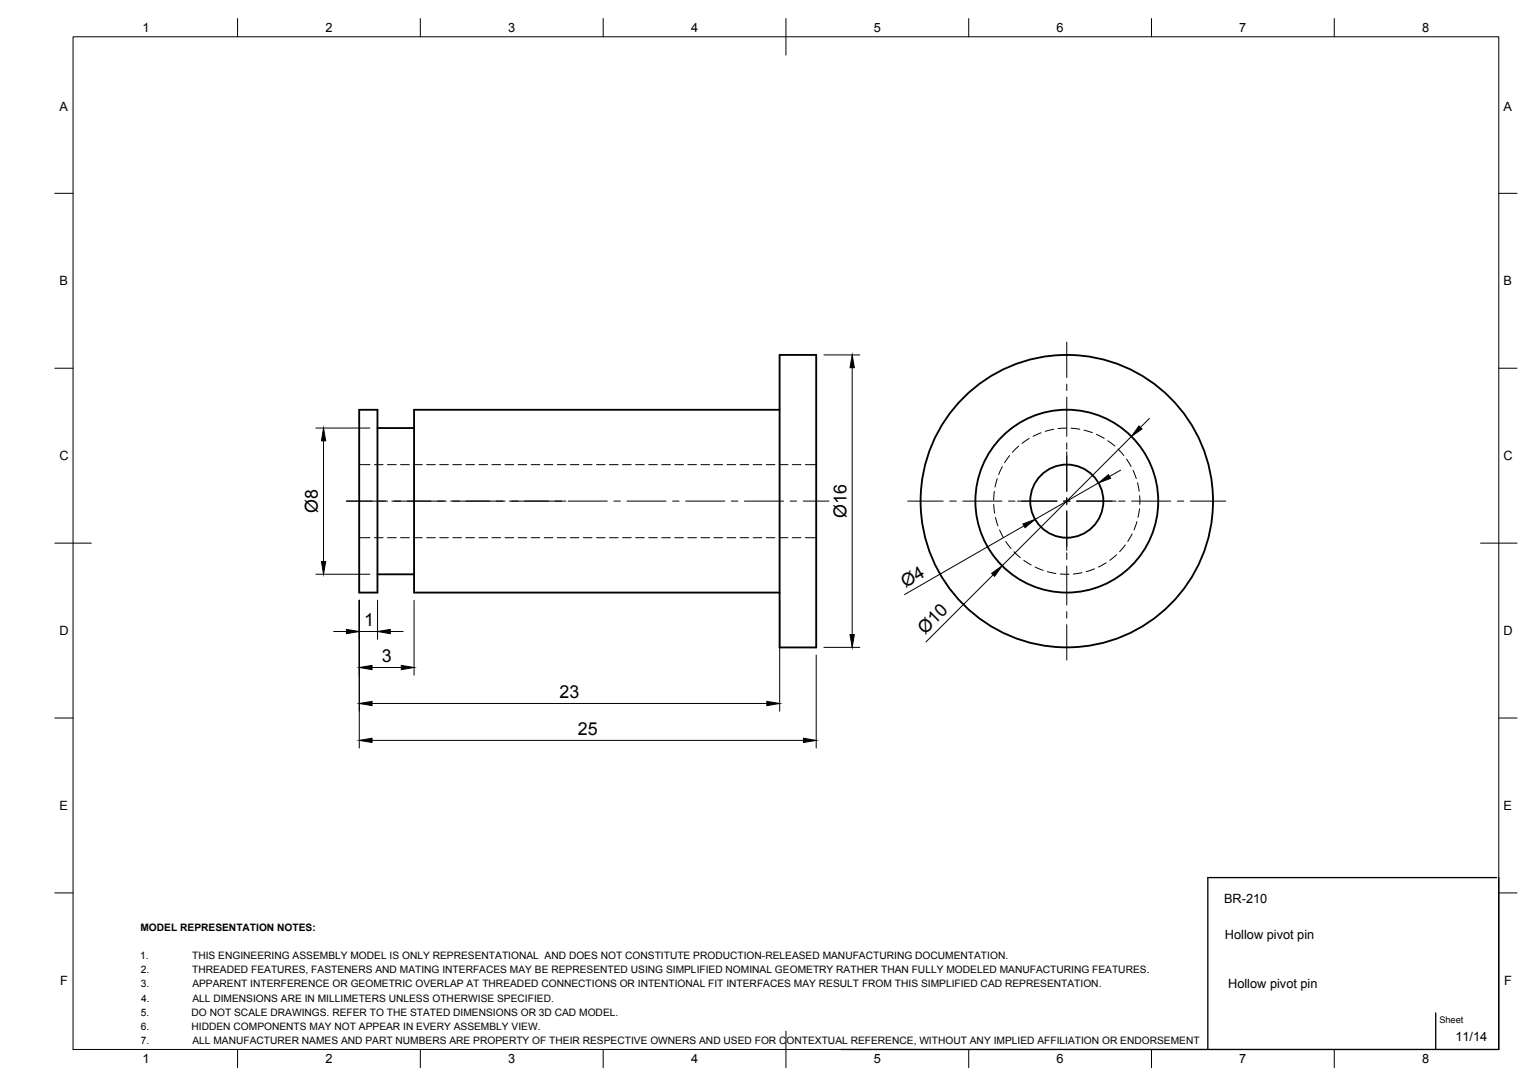
ISO-10303-21;
HEADER;
/* Generated by software containing ST-Developer
 * from STEP Tools, Inc. (www.steptools.com) 
 */

FILE_DESCRIPTION(
/* description */ ('Independent 1:2 reduction pantograph. 120 mm parallelogram sides; fix
ed fulcrum on the extension of a 240 mm link. Drawing point halfway al
ong its link, so its XY displacement is one half of the tracing point.
 Replaceable pivot bushes and retained pins. Calibration and productio
n accuracy unassigned.'),
/* implementation_level */ '2;1');

FILE_NAME(
/* name */ 'Hollow pivot pin.step',
/* time_stamp */ '2026-11-07T22:11:57-08:00',
/* author */ (''),
/* organization */ (''),
/* preprocessor_version */ 'ST-DEVELOPER v20.2',
/* originating_system */ 'Autodesk Translation Framework v15.17.0.0',
/* authorisation */ '');

FILE_SCHEMA (('AUTOMOTIVE_DESIGN { 1 0 10303 214 3 1 1 }'));
ENDSEC;

DATA;
#10=MECHANICAL_DESIGN_GEOMETRIC_PRESENTATION_REPRESENTATION('',(#191),#2926);
#165=SHAPE_REPRESENTATION_RELATIONSHIP('SRR','None',#3002,#178);
#178=ADVANCED_BREP_SHAPE_REPRESENTATION('',(#204),#2918);
#191=STYLED_ITEM('',(#3075),#204);
#204=MANIFOLD_SOLID_BREP('Body1',#1546);
#239=FACE_BOUND('',#468,.T.);
#240=FACE_BOUND('',#470,.T.);
#241=FACE_BOUND('',#473,.T.);
#242=FACE_BOUND('',#476,.T.);
#243=FACE_BOUND('',#480,.T.);
#279=PLANE('',#1792);
#280=PLANE('',#1794);
#281=PLANE('',#1798);
#282=PLANE('',#1803);
#283=PLANE('',#1808);
#347=FACE_OUTER_BOUND('',#466,.T.);
#348=FACE_OUTER_BOUND('',#467,.T.);
#349=FACE_OUTER_BOUND('',#469,.T.);
#350=FACE_OUTER_BOUND('',#471,.T.);
#351=FACE_OUTER_BOUND('',#472,.T.);
#352=FACE_OUTER_BOUND('',#474,.T.);
#353=FACE_OUTER_BOUND('',#475,.T.);
#354=FACE_OUTER_BOUND('',#477,.T.);
#355=FACE_OUTER_BOUND('',#478,.T.);
#356=FACE_OUTER_BOUND('',#479,.T.);
#466=EDGE_LOOP('',(#1241,#1242,#1243,#1244));
#467=EDGE_LOOP('',(#1245));
#468=EDGE_LOOP('',(#1246));
#469=EDGE_LOOP('',(#1247));
#470=EDGE_LOOP('',(#1248));
#471=EDGE_LOOP('',(#1249,#1250,#1251,#1252));
#472=EDGE_LOOP('',(#1253));
#473=EDGE_LOOP('',(#1254));
#474=EDGE_LOOP('',(#1255,#1256,#1257,#1258));
#475=EDGE_LOOP('',(#1259));
#476=EDGE_LOOP('',(#1260));
#477=EDGE_LOOP('',(#1261,#1262,#1263,#1264));
#478=EDGE_LOOP('',(#1265,#1266,#1267,#1268));
#479=EDGE_LOOP('',(#1269));
#480=EDGE_LOOP('',(#1270));
#580=LINE('',#2670,#661);
#581=LINE('',#2681,#662);
#582=LINE('',#2689,#663);
#583=LINE('',#2697,#664);
#584=LINE('',#2699,#665);
#661=VECTOR('',#2160,4.);
#662=VECTOR('',#2175,5.);
#663=VECTOR('',#2184,8.);
#664=VECTOR('',#2195,2.);
#665=VECTOR('',#2198,5.);
#739=CIRCLE('',#1790,4.);
#740=CIRCLE('',#1791,4.);
#741=CIRCLE('',#1793,5.);
#742=CIRCLE('',#1795,5.);
#743=CIRCLE('',#1797,5.);
#744=CIRCLE('',#1799,8.);
#745=CIRCLE('',#1800,5.);
#746=CIRCLE('',#1802,8.);
#747=CIRCLE('',#1804,2.);
#748=CIRCLE('',#1806,2.);
#843=VERTEX_POINT('',#2667);
#844=VERTEX_POINT('',#2669);
#845=VERTEX_POINT('',#2673);
#846=VERTEX_POINT('',#2676);
#847=VERTEX_POINT('',#2679);
#848=VERTEX_POINT('',#2683);
#849=VERTEX_POINT('',#2685);
#850=VERTEX_POINT('',#2688);
#851=VERTEX_POINT('',#2692);
#852=VERTEX_POINT('',#2695);
#985=EDGE_CURVE('',#843,#843,#739,.T.);
#986=EDGE_CURVE('',#843,#844,#580,.T.);
#987=EDGE_CURVE('',#844,#844,#740,.T.);
#988=EDGE_CURVE('',#845,#845,#741,.T.);
#989=EDGE_CURVE('',#846,#846,#742,.T.);
#990=EDGE_CURVE('',#847,#847,#743,.T.);
#991=EDGE_CURVE('',#847,#846,#581,.T.);
#992=EDGE_CURVE('',#848,#848,#744,.T.);
#993=EDGE_CURVE('',#849,#849,#745,.T.);
#994=EDGE_CURVE('',#848,#850,#582,.T.);
#995=EDGE_CURVE('',#850,#850,#746,.T.);
#996=EDGE_CURVE('',#851,#851,#747,.T.);
#997=EDGE_CURVE('',#852,#852,#748,.T.);
#998=EDGE_CURVE('',#852,#851,#583,.T.);
#999=EDGE_CURVE('',#845,#849,#584,.T.);
#1241=ORIENTED_EDGE('',*,*,#985,.T.);
#1242=ORIENTED_EDGE('',*,*,#986,.T.);
#1243=ORIENTED_EDGE('',*,*,#987,.F.);
#1244=ORIENTED_EDGE('',*,*,#986,.F.);
#1245=ORIENTED_EDGE('',*,*,#988,.F.);
#1246=ORIENTED_EDGE('',*,*,#985,.F.);
#1247=ORIENTED_EDGE('',*,*,#989,.F.);
#1248=ORIENTED_EDGE('',*,*,#987,.T.);
#1249=ORIENTED_EDGE('',*,*,#990,.F.);
#1250=ORIENTED_EDGE('',*,*,#991,.T.);
#1251=ORIENTED_EDGE('',*,*,#989,.T.);
#1252=ORIENTED_EDGE('',*,*,#991,.F.);
#1253=ORIENTED_EDGE('',*,*,#992,.T.);
#1254=ORIENTED_EDGE('',*,*,#993,.F.);
#1255=ORIENTED_EDGE('',*,*,#992,.F.);
#1256=ORIENTED_EDGE('',*,*,#994,.T.);
#1257=ORIENTED_EDGE('',*,*,#995,.T.);
#1258=ORIENTED_EDGE('',*,*,#994,.F.);
#1259=ORIENTED_EDGE('',*,*,#995,.F.);
#1260=ORIENTED_EDGE('',*,*,#996,.F.);
#1261=ORIENTED_EDGE('',*,*,#997,.F.);
#1262=ORIENTED_EDGE('',*,*,#998,.T.);
#1263=ORIENTED_EDGE('',*,*,#996,.T.);
#1264=ORIENTED_EDGE('',*,*,#998,.F.);
#1265=ORIENTED_EDGE('',*,*,#988,.T.);
#1266=ORIENTED_EDGE('',*,*,#999,.T.);
#1267=ORIENTED_EDGE('',*,*,#993,.T.);
#1268=ORIENTED_EDGE('',*,*,#999,.F.);
#1269=ORIENTED_EDGE('',*,*,#990,.T.);
#1270=ORIENTED_EDGE('',*,*,#997,.T.);
#1426=CYLINDRICAL_SURFACE('',#1789,4.);
#1427=CYLINDRICAL_SURFACE('',#1796,5.);
#1428=CYLINDRICAL_SURFACE('',#1801,8.);
#1429=CYLINDRICAL_SURFACE('',#1805,2.);
#1430=CYLINDRICAL_SURFACE('',#1807,5.);
#1491=ADVANCED_FACE('',(#347),#1426,.T.);
#1492=ADVANCED_FACE('',(#348,#239),#279,.F.);
#1493=ADVANCED_FACE('',(#349,#240),#280,.F.);
#1494=ADVANCED_FACE('',(#350),#1427,.T.);
#1495=ADVANCED_FACE('',(#351,#241),#281,.T.);
#1496=ADVANCED_FACE('',(#352),#1428,.T.);
#1497=ADVANCED_FACE('',(#353,#242),#282,.F.);
#1498=ADVANCED_FACE('',(#354),#1429,.F.);
#1499=ADVANCED_FACE('',(#355),#1430,.T.);
#1500=ADVANCED_FACE('',(#356,#243),#283,.T.);
#1546=CLOSED_SHELL('',(#1491,#1492,#1493,#1494,#1495,#1496,#1497,#1498,
#1499,#1500));
#1788=AXIS2_PLACEMENT_3D('',#2665,#2154,#2155);
#1789=AXIS2_PLACEMENT_3D('',#2666,#2156,#2157);
#1790=AXIS2_PLACEMENT_3D('',#2668,#2158,#2159);
#1791=AXIS2_PLACEMENT_3D('',#2671,#2161,#2162);
#1792=AXIS2_PLACEMENT_3D('',#2672,#2163,#2164);
#1793=AXIS2_PLACEMENT_3D('',#2674,#2165,#2166);
#1794=AXIS2_PLACEMENT_3D('',#2675,#2167,#2168);
#1795=AXIS2_PLACEMENT_3D('',#2677,#2169,#2170);
#1796=AXIS2_PLACEMENT_3D('',#2678,#2171,#2172);
#1797=AXIS2_PLACEMENT_3D('',#2680,#2173,#2174);
#1798=AXIS2_PLACEMENT_3D('',#2682,#2176,#2177);
#1799=AXIS2_PLACEMENT_3D('',#2684,#2178,#2179);
#1800=AXIS2_PLACEMENT_3D('',#2686,#2180,#2181);
#1801=AXIS2_PLACEMENT_3D('',#2687,#2182,#2183);
#1802=AXIS2_PLACEMENT_3D('',#2690,#2185,#2186);
#1803=AXIS2_PLACEMENT_3D('',#2691,#2187,#2188);
#1804=AXIS2_PLACEMENT_3D('',#2693,#2189,#2190);
#1805=AXIS2_PLACEMENT_3D('',#2694,#2191,#2192);
#1806=AXIS2_PLACEMENT_3D('',#2696,#2193,#2194);
#1807=AXIS2_PLACEMENT_3D('',#2698,#2196,#2197);
#1808=AXIS2_PLACEMENT_3D('',#2700,#2199,#2200);
#2154=DIRECTION('axis',(0.,0.,1.));
#2155=DIRECTION('refdir',(1.,0.,0.));
#2156=DIRECTION('center_axis',(0.,0.,1.));
#2157=DIRECTION('ref_axis',(1.,0.,0.));
#2158=DIRECTION('center_axis',(0.,0.,1.));
#2159=DIRECTION('ref_axis',(1.,0.,0.));
#2160=DIRECTION('',(0.,0.,1.));
#2161=DIRECTION('center_axis',(0.,0.,1.));
#2162=DIRECTION('ref_axis',(1.,0.,0.));
#2163=DIRECTION('center_axis',(0.,0.,-1.));
#2164=DIRECTION('ref_axis',(-1.,0.,0.));
#2165=DIRECTION('center_axis',(0.,0.,-1.));
#2166=DIRECTION('ref_axis',(1.,0.,0.));
#2167=DIRECTION('center_axis',(0.,0.,1.));
#2168=DIRECTION('ref_axis',(1.,0.,0.));
#2169=DIRECTION('center_axis',(0.,0.,1.));
#2170=DIRECTION('ref_axis',(1.,0.,0.));
#2171=DIRECTION('center_axis',(0.,0.,1.));
#2172=DIRECTION('ref_axis',(1.,0.,0.));
#2173=DIRECTION('center_axis',(0.,0.,1.));
#2174=DIRECTION('ref_axis',(1.,0.,0.));
#2175=DIRECTION('',(0.,0.,-1.));
#2176=DIRECTION('center_axis',(0.,0.,1.));
#2177=DIRECTION('ref_axis',(1.,0.,0.));
#2178=DIRECTION('center_axis',(0.,0.,1.));
#2179=DIRECTION('ref_axis',(1.,0.,0.));
#2180=DIRECTION('center_axis',(0.,0.,1.));
#2181=DIRECTION('ref_axis',(1.,0.,0.));
#2182=DIRECTION('center_axis',(0.,0.,1.));
#2183=DIRECTION('ref_axis',(1.,0.,0.));
#2184=DIRECTION('',(0.,0.,-1.));
#2185=DIRECTION('center_axis',(0.,0.,1.));
#2186=DIRECTION('ref_axis',(1.,0.,0.));
#2187=DIRECTION('center_axis',(0.,0.,1.));
#2188=DIRECTION('ref_axis',(1.,0.,0.));
#2189=DIRECTION('center_axis',(0.,0.,-1.));
#2190=DIRECTION('ref_axis',(1.,0.,0.));
#2191=DIRECTION('center_axis',(0.,0.,1.));
#2192=DIRECTION('ref_axis',(1.,0.,0.));
#2193=DIRECTION('center_axis',(0.,0.,-1.));
#2194=DIRECTION('ref_axis',(1.,0.,0.));
#2195=DIRECTION('',(0.,0.,-1.));
#2196=DIRECTION('center_axis',(0.,0.,1.));
#2197=DIRECTION('ref_axis',(1.,0.,0.));
#2198=DIRECTION('',(0.,0.,-1.));
#2199=DIRECTION('center_axis',(0.,0.,1.));
#2200=DIRECTION('ref_axis',(1.,0.,0.));
#2665=CARTESIAN_POINT('',(0.,0.,0.));
#2666=CARTESIAN_POINT('Origin',(0.,0.,21.));
#2667=CARTESIAN_POINT('',(-4.,-4.89858719658941E-16,20.));
#2668=CARTESIAN_POINT('Origin',(0.,0.,20.));
#2669=CARTESIAN_POINT('',(-4.,-4.89858719658941E-16,22.));
#2670=CARTESIAN_POINT('',(-4.,-4.89858719658941E-16,21.));
#2671=CARTESIAN_POINT('Origin',(0.,0.,22.));
#2672=CARTESIAN_POINT('Origin',(8.,0.,20.));
#2673=CARTESIAN_POINT('',(-5.,6.12323399573677E-16,20.));
#2674=CARTESIAN_POINT('Origin',(0.,0.,20.));
#2675=CARTESIAN_POINT('Origin',(4.,0.,22.));
#2676=CARTESIAN_POINT('',(-5.,-6.12323399573677E-16,22.));
#2677=CARTESIAN_POINT('Origin',(0.,0.,22.));
#2678=CARTESIAN_POINT('Origin',(0.,0.,0.));
#2679=CARTESIAN_POINT('',(-5.,-6.12323399573677E-16,23.));
#2680=CARTESIAN_POINT('Origin',(0.,0.,23.));
#2681=CARTESIAN_POINT('',(-5.,-6.12323399573677E-16,0.));
#2682=CARTESIAN_POINT('Origin',(0.,0.,0.));
#2683=CARTESIAN_POINT('',(-8.,-9.79717439317883E-16,0.));
#2684=CARTESIAN_POINT('Origin',(0.,0.,0.));
#2685=CARTESIAN_POINT('',(-5.,-6.12323399573677E-16,0.));
#2686=CARTESIAN_POINT('Origin',(0.,0.,0.));
#2687=CARTESIAN_POINT('Origin',(0.,0.,-2.));
#2688=CARTESIAN_POINT('',(-8.,-9.79717439317883E-16,-2.));
#2689=CARTESIAN_POINT('',(-8.,-9.79717439317883E-16,-2.));
#2690=CARTESIAN_POINT('Origin',(0.,0.,-2.));
#2691=CARTESIAN_POINT('Origin',(0.,0.,-2.));
#2692=CARTESIAN_POINT('',(-2.,-2.44929359829471E-16,-2.));
#2693=CARTESIAN_POINT('Origin',(0.,0.,-2.));
#2694=CARTESIAN_POINT('Origin',(0.,0.,0.));
#2695=CARTESIAN_POINT('',(-2.,-2.44929359829471E-16,23.));
#2696=CARTESIAN_POINT('Origin',(0.,0.,23.));
#2697=CARTESIAN_POINT('',(-2.,-2.44929359829471E-16,0.));
#2698=CARTESIAN_POINT('Origin',(0.,0.,0.));
#2699=CARTESIAN_POINT('',(-5.,-6.12323399573677E-16,0.));
#2700=CARTESIAN_POINT('Origin',(0.,0.,23.));
#2903=UNCERTAINTY_MEASURE_WITH_UNIT(LENGTH_MEASURE(0.01),#2927,
'DISTANCE_ACCURACY_VALUE',
'Maximum model space distance between geometric entities at asserted c
onnectivities');
#2911=UNCERTAINTY_MEASURE_WITH_UNIT(LENGTH_MEASURE(0.01),#2927,
'DISTANCE_ACCURACY_VALUE',
'Maximum model space distance between geometric entities at asserted c
onnectivities');
#2918=(
GEOMETRIC_REPRESENTATION_CONTEXT(3)
GLOBAL_UNCERTAINTY_ASSIGNED_CONTEXT((#2903))
GLOBAL_UNIT_ASSIGNED_CONTEXT((#2927,#2929,#2930))
REPRESENTATION_CONTEXT('','3D')
);
#2926=(
GEOMETRIC_REPRESENTATION_CONTEXT(3)
GLOBAL_UNCERTAINTY_ASSIGNED_CONTEXT((#2911))
GLOBAL_UNIT_ASSIGNED_CONTEXT((#2927,#2929,#2930))
REPRESENTATION_CONTEXT('','3D')
);
#2927=(
LENGTH_UNIT()
NAMED_UNIT(*)
SI_UNIT(.MILLI.,.METRE.)
);
#2929=(
NAMED_UNIT(*)
PLANE_ANGLE_UNIT()
SI_UNIT($,.RADIAN.)
);
#2930=(
NAMED_UNIT(*)
SI_UNIT($,.STERADIAN.)
SOLID_ANGLE_UNIT()
);
#2937=SHAPE_DEFINITION_REPRESENTATION(#2951,#3002);
#2951=PRODUCT_DEFINITION_SHAPE('',$,#3017);
#3002=SHAPE_REPRESENTATION('',(#1788),#2918);
#3010=PRODUCT_DEFINITION_CONTEXT('part definition',#3054,'design');
#3017=PRODUCT_DEFINITION('Hollow pivot pin','Hollow pivot pin',#3031,#3010);
#3031=PRODUCT_DEFINITION_FORMATION('',$,#3062);
#3054=APPLICATION_CONTEXT(
'Core Data for Automotive Mechanical Design Process');
#3055=PRODUCT_CONTEXT('part definition',#3054,'mechanical');
#3062=PRODUCT('Hollow pivot pin','Hollow pivot pin',$,(#3055));
#3075=PRESENTATION_STYLE_ASSIGNMENT((#3087));
#3087=SURFACE_STYLE_USAGE(.BOTH.,#3099);
#3099=SURFACE_SIDE_STYLE('',(#3111));
#3111=SURFACE_STYLE_FILL_AREA(#3123);
#3123=FILL_AREA_STYLE('Pivot gray',(#3135));
#3135=FILL_AREA_STYLE_COLOUR('Pivot gray',#3147);
#3147=COLOUR_RGB('Pivot gray',0.407843137254902,0.447058823529412,0.498039215686275);
ENDSEC;
END-ISO-10303-21;
